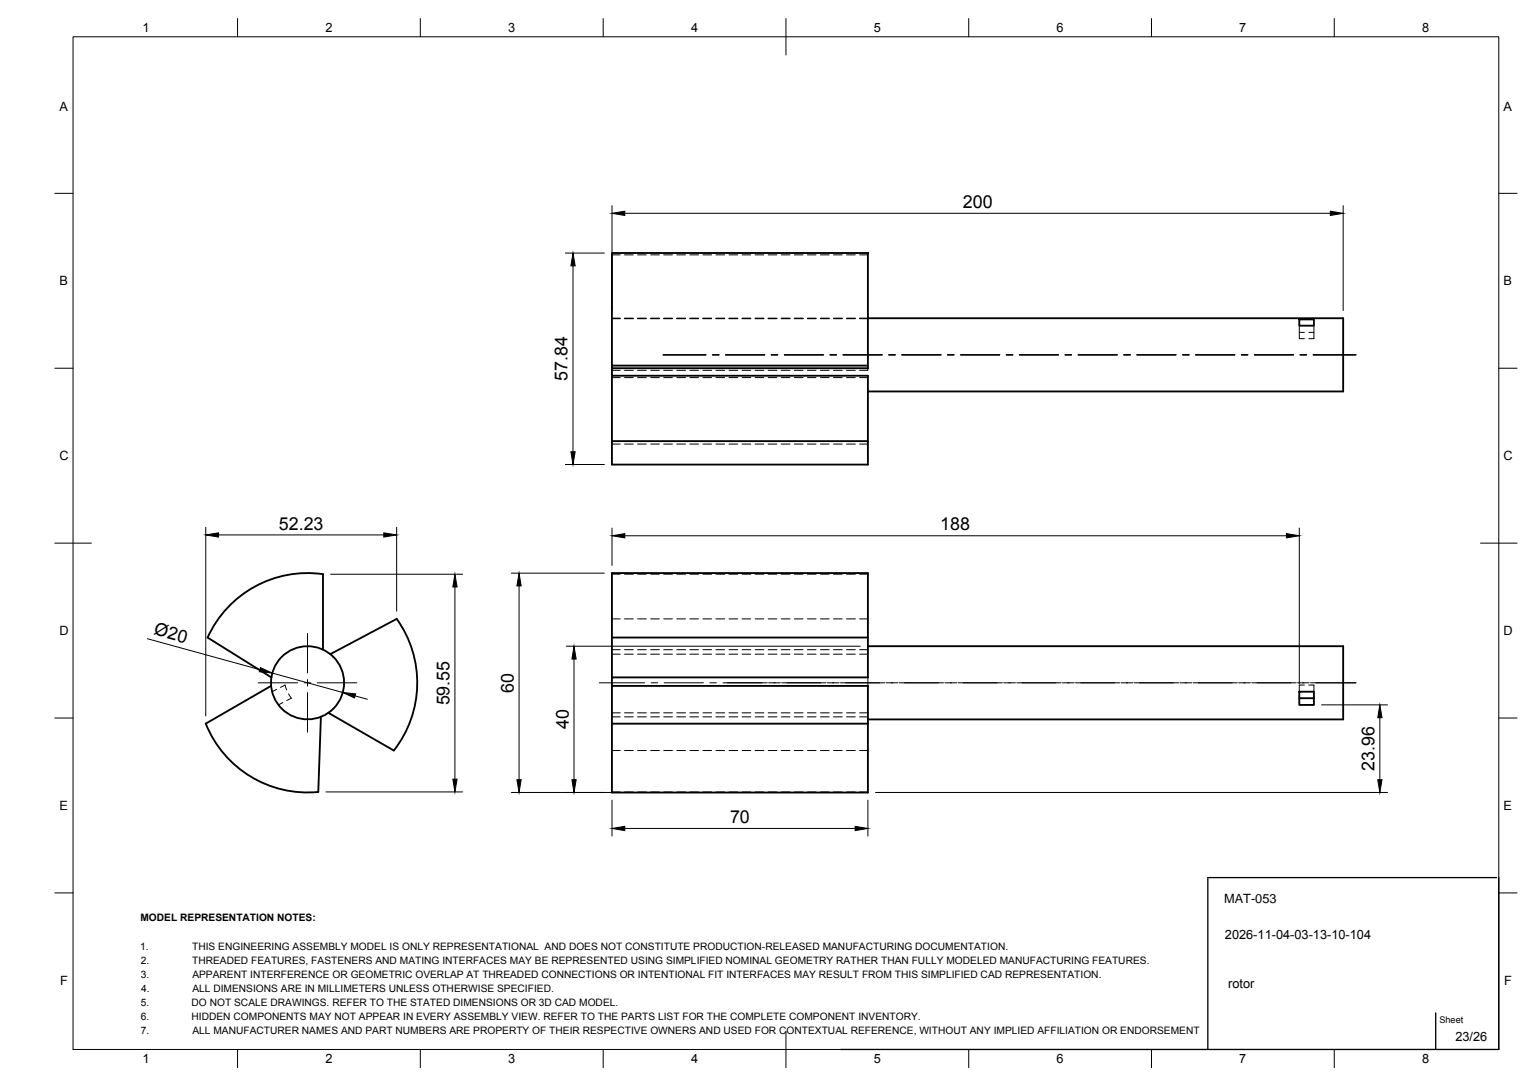
ISO-10303-21;
HEADER;
FILE_DESCRIPTION (('STEP AP214'),
    '1' );
FILE_NAME ('rotor.step',
    '2026-10-10T03:43:58',
    ( '' ),
    ( '' ),
    'SwSTEP 2.0',
    'SolidWorks 2026',
    '' );
FILE_SCHEMA (( 'AUTOMOTIVE_DESIGN' ));
ENDSEC;

DATA;
#17=CARTESIAN_POINT ( 'NONE',  ( 0.000000000000000000, 70.00000000000000000, 0.000000000000000000 ) ) ;
#158=VECTOR ( 'NONE', #16298, 1000.000000000000000 ) ;
#309=LINE ( 'NONE', #37951, #56611 ) ;
#450=VECTOR ( 'NONE', #55912, 1000.000000000000000 ) ;
#456=COLOUR_RGB ( '',0.7921568627450980005, 0.8196078431372548767, 0.9333333333333333481 ) ;
#467=CIRCLE ( 'NONE', #25205, 10.00000000000000000 ) ;
#513=( NAMED_UNIT ( * ) PLANE_ANGLE_UNIT ( ) SI_UNIT ( $, .RADIAN. ) );
#637=ORIENTED_EDGE ( 'NONE', *, *, #53348, .T. ) ;
#947=CARTESIAN_POINT ( 'NONE',  ( 0.000000000000000000, 70.00000000000000000, 0.000000000000000000 ) ) ;
#1209=EDGE_CURVE ( 'NONE', #16807, #23774, #1533, .T. ) ;
#1274=FACE_OUTER_BOUND ( 'NONE', #43238, .T. ) ;
#1425=AXIS2_PLACEMENT_3D ( 'NONE', #25627, #58986, #15401 ) ;
#1533=LINE ( 'NONE', #38469, #44099 ) ;
#1588=CARTESIAN_POINT ( 'NONE',  ( -12.50012419267789454, 70.00000000000000000, -27.27172336262650987 ) ) ;
#1598=FACE_OUTER_BOUND ( 'NONE', #21651, .T. ) ;
#1621=CARTESIAN_POINT ( 'NONE',  ( 0.000000000000000000, 200.0000000000000000, 0.000000000000000000 ) ) ;
#1632=ORIENTED_EDGE ( 'NONE', *, *, #41608, .F. ) ;
#1645=ORIENTED_EDGE ( 'NONE', *, *, #47561, .T. ) ;
#1859=VERTEX_POINT ( 'NONE', #41000 ) ;
#1935=AXIS2_PLACEMENT_3D ( 'NONE', #55616, #50350, #54908 ) ;
#2096=ORIENTED_EDGE ( 'NONE', *, *, #47172, .F. ) ;
#2200=CARTESIAN_POINT ( 'NONE',  ( 0.000000000000000000, 0.000000000000000000, 0.000000000000000000 ) ) ;
#2470=PLANE ( 'NONE',  #7800 ) ;
#2490=PLANE ( 'NONE',  #35776 ) ;
#2533=CIRCLE ( 'NONE', #56453, 30.00000000000000000 ) ;
#2546=ORIENTED_EDGE ( 'NONE', *, *, #59775, .T. ) ;
#2559=EDGE_LOOP ( 'NONE', ( #62181, #13017, #69406, #67367 ) ) ;
#2584=ORIENTED_EDGE ( 'NONE', *, *, #47172, .T. ) ;
#2625=ORIENTED_EDGE ( 'NONE', *, *, #31517, .T. ) ;
#2755=FACE_BOUND ( 'NONE', #28802, .T. ) ;
#2940=CARTESIAN_POINT ( 'NONE',  ( 9.737557066527559257, 192.0000000000000000, 2.275957463600584596 ) ) ;
#3029=EDGE_CURVE ( 'NONE', #41495, #19589, #60995, .T. ) ;
#3127=VECTOR ( 'NONE', #17134, 1000.000000000000000 ) ;
#3205=EDGE_CURVE ( 'NONE', #15244, #53408, #69376, .T. ) ;
#3229=CIRCLE ( 'NONE', #31340, 30.00000000000000000 ) ;
#3559=ADVANCED_FACE ( 'NONE', ( #18572 ), #60439, .F. ) ;
#3584=CYLINDRICAL_SURFACE ( 'NONE', #18065, 30.00000000000000000 ) ;
#3606=DIRECTION ( 'NONE',  ( -0.000000000000000000, 1.000000000000000000, 0.000000000000000000 ) ) ;
#3647=FACE_OUTER_BOUND ( 'NONE', #22136, .T. ) ;
#3725=( GEOMETRIC_REPRESENTATION_CONTEXT ( 3 ) GLOBAL_UNCERTAINTY_ASSIGNED_CONTEXT ( ( #66987 ) ) GLOBAL_UNIT_ASSIGNED_CONTEXT ( ( #56756, #15223, #36690 ) ) REPRESENTATION_CONTEXT ( 'NONE', 'WORKASPACE' ) );
#3943=DIRECTION ( 'NONE',  ( -0.8410447872859948548, 0.000000000000000000, 0.5409654940743040541 ) ) ;
#3944=AXIS2_PLACEMENT_3D ( 'NONE', #67199, #40779, #62236 ) ;
#3990=VECTOR ( 'NONE', #9870, 1000.000000000000000 ) ;
#4513=DIRECTION ( 'NONE',  ( 0.000000000000000000, 0.000000000000000000, -1.000000000000000000 ) ) ;
#4695=CARTESIAN_POINT ( 'NONE',  ( 9.737557066527559257, 188.0000000000000000, 2.275957463600585040 ) ) ;
#4837=CARTESIAN_POINT ( 'NONE',  ( 0.2033771190674383833, 0.000000000000000000, 4.235016458833691821 ) ) ;
#4881=VECTOR ( 'NONE', #9082, 1000.000000000000114 ) ;
#5095=ORIENTED_EDGE ( 'NONE', *, *, #20108, .T. ) ;
#5142=DIRECTION ( 'NONE',  ( 0.000000000000000000, 0.000000000000000000, -1.000000000000000000 ) ) ;
#5186=VECTOR ( 'NONE', #48521, 1000.000000000000000 ) ;
#5268=EDGE_CURVE ( 'NONE', #22494, #32164, #467, .T. ) ;
#5688=AXIS2_PLACEMENT_3D ( 'NONE', #62242, #23924, #39755 ) ;
#5807=PLANE ( 'NONE',  #12101 ) ;
#5820=FACE_OUTER_BOUND ( 'NONE', #11195, .T. ) ;
#5922=CIRCLE ( 'NONE', #32905, 10.00000000000000000 ) ;
#5931=EDGE_CURVE ( 'NONE', #43885, #57004, #38522, .T. ) ;
#5947=FACE_OUTER_BOUND ( 'NONE', #36620, .T. ) ;
#6067=ORIENTED_EDGE ( 'NONE', *, *, #59775, .F. ) ;
#6088=ORIENTED_EDGE ( 'NONE', *, *, #65385, .T. ) ;
#6211=CARTESIAN_POINT ( 'NONE',  ( 9.737557066527559257, 192.0000000000000000, 2.275957463600585040 ) ) ;
#6261=LINE ( 'NONE', #28414, #36185 ) ;
#6269=EDGE_CURVE ( 'NONE', #24463, #24269, #18512, .T. ) ;
#6455=EDGE_CURVE ( 'NONE', #24735, #28455, #61192, .T. ) ;
#6554=DIRECTION ( 'NONE',  ( 0.000000000000000000, -0.000000000000000000, 1.000000000000000000 ) ) ;
#6584=EDGE_CURVE ( 'NONE', #24735, #41495, #13935, .T. ) ;
#6671=CARTESIAN_POINT ( 'NONE',  ( -9.119248870808011276, 0.000000000000000000, 4.103571619000548232 ) ) ;
#6698=CARTESIAN_POINT ( 'NONE',  ( -17.36794314067741496, 70.00000000000000000, 24.46128678263259815 ) ) ;
#6858=ORIENTED_EDGE ( 'NONE', *, *, #8268, .F. ) ;
#7138=VECTOR ( 'NONE', #50452, 1000.000000000000000 ) ;
#7268=VECTOR ( 'NONE', #48702, 1000.000000000000000 ) ;
#7376=EDGE_LOOP ( 'NONE', ( #17858, #25912, #30020, #37099 ) ) ;
#7467=CARTESIAN_POINT ( 'NONE',  ( 18.62350602913453201, 0.000000000000000000, 23.51946052065798298 ) ) ;
#7577=CARTESIAN_POINT ( 'NONE',  ( 0.000000000000000000, 0.000000000000000000, 0.000000000000000000 ) ) ;
#7619=VERTEX_POINT ( 'NONE', #18144 ) ;
#7684=ORIENTED_EDGE ( 'NONE', *, *, #20480, .T. ) ;
#7800=AXIS2_PLACEMENT_3D ( 'NONE', #47017, #41741, #61888 ) ;
#7829=CYLINDRICAL_SURFACE ( 'NONE', #28638, 30.00000000000000000 ) ;
#7957=DIRECTION ( 'NONE',  ( -0.000000000000000000, 1.000000000000000000, -0.000000000000000000 ) ) ;
#8251=ORIENTED_EDGE ( 'NONE', *, *, #19759, .T. ) ;
#8268=EDGE_CURVE ( 'NONE', #8643, #36732, #63662, .T. ) ;
#8319=DIRECTION ( 'NONE',  ( 1.000000000000000000, 0.000000000000000000, 0.000000000000000000 ) ) ;
#8362=MECHANICAL_DESIGN_GEOMETRIC_PRESENTATION_REPRESENTATION('',(#39786),#3725);
#8384=DIRECTION ( 'NONE',  ( -0.000000000000000000, -1.000000000000000000, -0.000000000000000000 ) ) ;
#8517=CARTESIAN_POINT ( 'NONE',  ( 1.224646799147353256E-15, 200.0000000000000000, 10.00000000000000000 ) ) ;
#8543=VERTEX_POINT ( 'NONE', #25611 ) ;
#8643=VERTEX_POINT ( 'NONE', #67319 ) ;
#8758=LINE ( 'NONE', #29499, #68982 ) ;
#8847=PLANE ( 'NONE',  #53612 ) ;
#9082=DIRECTION ( 'NONE',  ( 0.4887922226926450509, 0.000000000000000000, -0.8724002309921654597 ) ) ;
#9354=AXIS2_PLACEMENT_3D ( 'NONE', #45077, #60911, #12734 ) ;
#9450=DIRECTION ( 'NONE',  ( 0.000000000000000000, -1.000000000000000000, 0.000000000000000000 ) ) ;
#9699=LINE ( 'NONE', #15316, #18300 ) ;
#9760=CARTESIAN_POINT ( 'NONE',  ( -9.119248870808011276, 70.00000000000000000, 4.103571619000548232 ) ) ;
#9806=CIRCLE ( 'NONE', #1935, 10.00000000000000000 ) ;
#9808=VERTEX_POINT ( 'NONE', #22364 ) ;
#9870=DIRECTION ( 'NONE',  ( 0.5111246509603011301, 0.000000000000000000, 0.8595065975201763298 ) ) ;
#9984=DIRECTION ( 'NONE',  ( 0.8660254037844433705, 0.000000000000000000, -0.4999999999999918954 ) ) ;
#10072=ORIENTED_EDGE ( 'NONE', *, *, #55049, .T. ) ;
#10118=LINE ( 'NONE', #4837, #34031 ) ;
#10295=AXIS2_PLACEMENT_3D ( 'NONE', #15592, #52853, #58479 ) ;
#10688=ORIENTED_EDGE ( 'NONE', *, *, #6269, .T. ) ;
#10694=AXIS2_PLACEMENT_3D ( 'NONE', #41357, #62809, #14614 ) ;
#10699=ORIENTED_EDGE ( 'NONE', *, *, #32324, .F. ) ;
#10743=FACE_OUTER_BOUND ( 'NONE', #34044, .T. ) ;
#10903=LINE ( 'NONE', #64367, #49186 ) ;
#10960=ADVANCED_FACE ( 'NONE', ( #1274 ), #17086, .T. ) ;
#11102=DIRECTION ( 'NONE',  ( -0.9999168736529502333, 0.000000000000000000, 0.01289363347198224652 ) ) ;
#11175=ORIENTED_EDGE ( 'NONE', *, *, #35410, .T. ) ;
#11187=VECTOR ( 'NONE', #67603, 1000.000000000000000 ) ;
#11195=EDGE_LOOP ( 'NONE', ( #43138, #50240, #35379, #36120, #11963, #1632, #41191, #63277, #68258, #42912 ) ) ;
#11806=( GEOMETRIC_REPRESENTATION_CONTEXT ( 3 ) GLOBAL_UNCERTAINTY_ASSIGNED_CONTEXT ( ( #39538 ) ) GLOBAL_UNIT_ASSIGNED_CONTEXT ( ( #37800, #513, #38141 ) ) REPRESENTATION_CONTEXT ( 'NONE', 'WORKASPACE' ) );
#11963=ORIENTED_EDGE ( 'NONE', *, *, #22370, .T. ) ;
#12101=AXIS2_PLACEMENT_3D ( 'NONE', #31864, #64208, #26585 ) ;
#12156=ORIENTED_EDGE ( 'NONE', *, *, #53282, .F. ) ;
#12160=CARTESIAN_POINT ( 'NONE',  ( -29.68020330876228385, 0.000000000000000000, 4.368699068434031219 ) ) ;
#12734=DIRECTION ( 'NONE',  ( 0.000000000000000000, 0.000000000000000000, -1.000000000000000000 ) ) ;
#12756=CARTESIAN_POINT ( 'NONE',  ( 0.000000000000000000, 70.00000000000000000, 0.000000000000000000 ) ) ;
#12971=DIRECTION ( 'NONE',  ( 0.000000000000000000, 0.000000000000000000, -1.000000000000000000 ) ) ;
#13017=ORIENTED_EDGE ( 'NONE', *, *, #59463, .T. ) ;
#13419=EDGE_CURVE ( 'NONE', #32766, #41495, #62864, .T. ) ;
#13492=DIRECTION ( 'NONE',  ( 0.000000000000000000, -0.000000000000000000, -1.000000000000000000 ) ) ;
#13577=DIRECTION ( 'NONE',  ( -0.000000000000000000, -1.000000000000000000, -0.000000000000000000 ) ) ;
#13604=ORIENTED_EDGE ( 'NONE', *, *, #22162, .F. ) ;
#13935=LINE ( 'NONE', #36782, #34286 ) ;
#13961=EDGE_CURVE ( 'NONE', #18376, #21875, #28435, .T. ) ;
#14150=PLANE ( 'NONE',  #20788 ) ;
#14262=ORIENTED_EDGE ( 'NONE', *, *, #52512, .F. ) ;
#14534=FILL_AREA_STYLE_COLOUR ( '', #456 ) ;
#14614=DIRECTION ( 'NONE',  ( 0.000000000000000000, 0.000000000000000000, -1.000000000000000000 ) ) ;
#14719=FACE_OUTER_BOUND ( 'NONE', #15340, .T. ) ;
#14822=VECTOR ( 'NONE', #60512, 1000.000000000000000 ) ;
#14870=SURFACE_STYLE_FILL_AREA ( #35991 ) ;
#14908=CARTESIAN_POINT ( 'NONE',  ( 9.737557066527559257, 188.0000000000000000, 2.275957463600584596 ) ) ;
#15042=ORIENTED_EDGE ( 'NONE', *, *, #54768, .T. ) ;
#15142=CARTESIAN_POINT ( 'NONE',  ( 18.62350602913453557, 70.00000000000000000, 23.51946052065799364 ) ) ;
#15180=EDGE_CURVE ( 'NONE', #57004, #9808, #53700, .T. ) ;
#15223=( NAMED_UNIT ( * ) PLANE_ANGLE_UNIT ( ) SI_UNIT ( $, .RADIAN. ) );
#15244=VERTEX_POINT ( 'NONE', #32268 ) ;
#15259=DIRECTION ( 'NONE',  ( 0.000000000000000000, -1.000000000000000000, 0.000000000000000000 ) ) ;
#15316=CARTESIAN_POINT ( 'NONE',  ( 0.000000000000000000, 200.0000000000000000, -10.00000000000000000 ) ) ;
#15340=EDGE_LOOP ( 'NONE', ( #65390, #64020, #51418, #38157 ) ) ;
#15401=DIRECTION ( 'NONE',  ( -1.000000000000000000, 0.000000000000000000, -0.000000000000000000 ) ) ;
#15472=CIRCLE ( 'NONE', #33452, 10.00000000000000000 ) ;
#15592=CARTESIAN_POINT ( 'NONE',  ( 9.737557066527559257, 200.0000000000000000, 2.275957463600584596 ) ) ;
#15661=DIRECTION ( 'NONE',  ( -0.000000000000000000, -1.000000000000000000, -0.000000000000000000 ) ) ;
#15663=DIRECTION ( 'NONE',  ( 0.000000000000000000, -1.000000000000000000, 0.000000000000000000 ) ) ;
#15702=VECTOR ( 'NONE', #66791, 1000.000000000000000 ) ;
#15713=ORIENTED_EDGE ( 'NONE', *, *, #6455, .T. ) ;
#16298=DIRECTION ( 'NONE',  ( -1.000000000000000000, 0.000000000000000000, 0.000000000000000000 ) ) ;
#16595=ORIENTED_EDGE ( 'NONE', *, *, #31517, .F. ) ;
#16661=ORIENTED_EDGE ( 'NONE', *, *, #59463, .F. ) ;
#16742=ORIENTED_EDGE ( 'NONE', *, *, #24162, .F. ) ;
#16807=VERTEX_POINT ( 'NONE', #53772 ) ;
#16822=ORIENTED_EDGE ( 'NONE', *, *, #45120, .T. ) ;
#16837=ORIENTED_EDGE ( 'NONE', *, *, #53571, .F. ) ;
#17075=AXIS2_PLACEMENT_3D ( 'NONE', #18933, #8384, #12971 ) ;
#17086=PLANE ( 'NONE',  #52536 ) ;
#17095=EDGE_LOOP ( 'NONE', ( #52386, #18112, #28006, #32395 ) ) ;
#17103=DIRECTION ( 'NONE',  ( -0.8660254037844362651, 0.000000000000000000, -0.5000000000000038858 ) ) ;
#17134=DIRECTION ( 'NONE',  ( -0.000000000000000000, 1.000000000000000000, -0.000000000000000000 ) ) ;
#17242=EDGE_LOOP ( 'NONE', ( #52824, #58022, #67424, #2546 ) ) ;
#17320=ORIENTED_EDGE ( 'NONE', *, *, #13419, .F. ) ;
#17348=DIRECTION ( 'NONE',  ( 0.000000000000000000, -1.000000000000000000, 0.000000000000000000 ) ) ;
#17365=VERTEX_POINT ( 'NONE', #28271 ) ;
#17466=CARTESIAN_POINT ( 'NONE',  ( -29.68020330876228030, 0.000000000000000000, 4.368699068434031219 ) ) ;
#17492=CARTESIAN_POINT ( 'NONE',  ( 1.224646799147353256E-15, 200.0000000000000000, 10.00000000000000000 ) ) ;
#17691=ORIENTED_EDGE ( 'NONE', *, *, #55587, .T. ) ;
#17858=ORIENTED_EDGE ( 'NONE', *, *, #53236, .F. ) ;
#17892=CARTESIAN_POINT ( 'NONE',  ( 0.000000000000000000, 70.00000000000000000, 0.000000000000000000 ) ) ;
#17900=DIRECTION ( 'NONE',  ( -1.000000000000000000, 0.000000000000000000, 0.000000000000000000 ) ) ;
#18009=CARTESIAN_POINT ( 'NONE',  ( 8.113421703707349053, 70.00000000000000000, 5.845715376051984435 ) ) ;
#18065=AXIS2_PLACEMENT_3D ( 'NONE', #46487, #58088, #27100 ) ;
#18112=ORIENTED_EDGE ( 'NONE', *, *, #3029, .F. ) ;
#18144=CARTESIAN_POINT ( 'NONE',  ( 29.86806733335506436, 70.00000000000000000, 2.810436579993893957 ) ) ;
#18265=EDGE_CURVE ( 'NONE', #27416, #21875, #30226, .T. ) ;
#18300=VECTOR ( 'NONE', #15661, 1000.000000000000000 ) ;
#18376=VERTEX_POINT ( 'NONE', #62581 ) ;
#18512=CIRCLE ( 'NONE', #48798, 30.00000000000000000 ) ;
#18572=FACE_OUTER_BOUND ( 'NONE', #17242, .T. ) ;
#18600=AXIS2_PLACEMENT_3D ( 'NONE', #43927, #54482, #27407 ) ;
#18683=FACE_OUTER_BOUND ( 'NONE', #37789, .T. ) ;
#18749=LINE ( 'NONE', #40207, #63574 ) ;
#18826=ORIENTED_EDGE ( 'NONE', *, *, #25756, .T. ) ;
#18933=CARTESIAN_POINT ( 'NONE',  ( 0.000000000000000000, 200.0000000000000000, 0.000000000000000000 ) ) ;
#18937=VERTEX_POINT ( 'NONE', #52862 ) ;
#19410=AXIS2_PLACEMENT_3D ( 'NONE', #49515, #34422, #38995 ) ;
#19489=CARTESIAN_POINT ( 'NONE',  ( 9.737557066527559257, 200.0000000000000000, 2.275957463600584596 ) ) ;
#19589=VERTEX_POINT ( 'NONE', #48358 ) ;
#19639=DIRECTION ( 'NONE',  ( -1.000000000000000000, 0.000000000000000000, 0.000000000000000000 ) ) ;
#19759=EDGE_CURVE ( 'NONE', #32766, #23774, #21564, .T. ) ;
#19928=ORIENTED_EDGE ( 'NONE', *, *, #69410, .T. ) ;
#20108=EDGE_CURVE ( 'NONE', #24269, #27416, #22180, .T. ) ;
#20308=ORIENTED_EDGE ( 'NONE', *, *, #22057, .F. ) ;
#20480=EDGE_CURVE ( 'NONE', #48193, #58381, #6261, .T. ) ;
#20490=PRESENTATION_STYLE_ASSIGNMENT (( #57446 ) ) ;
#20674=CARTESIAN_POINT ( 'NONE',  ( 5.737557066527558369, 188.0000000000000000, 2.275957463600585040 ) ) ;
#20778=LINE ( 'NONE', #31682, #5186 ) ;
#20788=AXIS2_PLACEMENT_3D ( 'NONE', #40529, #3943, #41914 ) ;
#20839=VERTEX_POINT ( 'NONE', #21757 ) ;
#21094=DIRECTION ( 'NONE',  ( -0.000000000000000000, 1.000000000000000000, -0.000000000000000000 ) ) ;
#21275=EDGE_LOOP ( 'NONE', ( #48937, #6067, #1645, #32059, #28609 ) ) ;
#21564=LINE ( 'NONE', #14908, #158 ) ;
#21575=EDGE_LOOP ( 'NONE', ( #62682, #36983, #35955, #40340 ) ) ;
#21651=EDGE_LOOP ( 'NONE', ( #54885, #45467, #21777, #2625 ) ) ;
#21757=CARTESIAN_POINT ( 'NONE',  ( -1.333402737265964699, 0.000000000000000000, -9.910703160737465822 ) ) ;
#21777=ORIENTED_EDGE ( 'NONE', *, *, #41837, .T. ) ;
#21783=PLANE ( 'NONE',  #18600 ) ;
#21875=VERTEX_POINT ( 'NONE', #31314 ) ;
#21940=EDGE_LOOP ( 'NONE', ( #16661, #20308, #15713, #38662 ) ) ;
#22049=AXIS2_PLACEMENT_3D ( 'NONE', #36182, #58313, #47406 ) ;
#22057=EDGE_CURVE ( 'NONE', #24735, #18937, #28447, .T. ) ;
#22098=DIRECTION ( 'NONE',  ( 0.4887922226926451064, 0.000000000000000000, -0.8724002309921654597 ) ) ;
#22136=EDGE_LOOP ( 'NONE', ( #66291, #30867, #17691, #8251 ) ) ;
#22162=EDGE_CURVE ( 'NONE', #24494, #1859, #36156, .T. ) ;
#22180=LINE ( 'NONE', #6698, #14822 ) ;
#22343=DIRECTION ( 'NONE',  ( 0.000000000000000000, -1.000000000000000000, 0.000000000000000000 ) ) ;
#22364=CARTESIAN_POINT ( 'NONE',  ( -1.333402737265964699, 70.00000000000000000, -9.910703160737465822 ) ) ;
#22370=EDGE_CURVE ( 'NONE', #20839, #9808, #56140, .T. ) ;
#22404=CARTESIAN_POINT ( 'NONE',  ( 0.000000000000000000, 0.000000000000000000, -10.00000000000000000 ) ) ;
#22494=VERTEX_POINT ( 'NONE', #32515 ) ;
#22749=DIRECTION ( 'NONE',  ( 0.000000000000000000, 0.000000000000000000, -1.000000000000000000 ) ) ;
#22869=VECTOR ( 'NONE', #41629, 999.9999999999998863 ) ;
#23387=SHAPE_REPRESENTATION_RELATIONSHIP ( 'NONE' , 'NONE' ,  #36174, #54154 ) ;
#23522=FACE_OUTER_BOUND ( 'NONE', #51607, .T. ) ;
#23700=PLANE ( 'NONE',  #27020 ) ;
#23774=VERTEX_POINT ( 'NONE', #20674 ) ;
#23924=DIRECTION ( 'NONE',  ( -0.000000000000000000, -1.000000000000000000, -0.000000000000000000 ) ) ;
#24027=VECTOR ( 'NONE', #7957, 1000.000000000000000 ) ;
#24094=DIRECTION ( 'NONE',  ( -0.000000000000000000, -1.000000000000000000, -0.000000000000000000 ) ) ;
#24162=EDGE_CURVE ( 'NONE', #48193, #8543, #33104, .T. ) ;
#24269=VERTEX_POINT ( 'NONE', #51147 ) ;
#24436=DIRECTION ( 'NONE',  ( 0.000000000000000000, -0.000000000000000000, 1.000000000000000000 ) ) ;
#24463=VERTEX_POINT ( 'NONE', #7467 ) ;
#24494=VERTEX_POINT ( 'NONE', #27859 ) ;
#24629=FACE_OUTER_BOUND ( 'NONE', #2559, .T. ) ;
#24659=CARTESIAN_POINT ( 'NONE',  ( -21.78980970457817179, 0.000000000000000000, 33.04664611826583354 ) ) ;
#24697=DIRECTION ( 'NONE',  ( 0.000000000000000000, -1.000000000000000000, 0.000000000000000000 ) ) ;
#24716=FACE_OUTER_BOUND ( 'NONE', #59779, .T. ) ;
#24735=VERTEX_POINT ( 'NONE', #52941 ) ;
#24816=ORIENTED_EDGE ( 'NONE', *, *, #24162, .T. ) ;
#25205=AXIS2_PLACEMENT_3D ( 'NONE', #34821, #52026, #41127 ) ;
#25405=ORIENTED_EDGE ( 'NONE', *, *, #53348, .F. ) ;
#25422=DIRECTION ( 'NONE',  ( 0.000000000000000000, -0.000000000000000000, -1.000000000000000000 ) ) ;
#25447=PRODUCT_DEFINITION_FORMATION_WITH_SPECIFIED_SOURCE ( 'ANY', '', #65900, .NOT_KNOWN. ) ;
#25470=LINE ( 'NONE', #46907, #22869 ) ;
#25576=ORIENTED_EDGE ( 'NONE', *, *, #60819, .T. ) ;
#25611=CARTESIAN_POINT ( 'NONE',  ( 9.249622075198342230, 70.00000000000000000, 3.800590936420744193 ) ) ;
#25627=CARTESIAN_POINT ( 'NONE',  ( 9.850262805259839993, 200.0000000000000000, -1.724042536399416070 ) ) ;
#25756=EDGE_CURVE ( 'NONE', #43631, #8543, #20778, .T. ) ;
#25829=DIRECTION ( 'NONE',  ( 0.000000000000000000, -1.000000000000000000, 0.000000000000000000 ) ) ;
#25843=ORIENTED_EDGE ( 'NONE', *, *, #5931, .F. ) ;
#25912=ORIENTED_EDGE ( 'NONE', *, *, #19759, .F. ) ;
#26222=CIRCLE ( 'NONE', #9354, 10.00000000000000000 ) ;
#26428=CIRCLE ( 'NONE', #10694, 10.00000000000000000 ) ;
#26442=ADVANCED_FACE ( 'NONE', ( #33863 ), #7829, .T. ) ;
#26585=DIRECTION ( 'NONE',  ( 0.000000000000000000, -0.000000000000000000, -1.000000000000000000 ) ) ;
#26601=CARTESIAN_POINT ( 'NONE',  ( 0.000000000000000000, 200.0000000000000000, 0.000000000000000000 ) ) ;
#26749=ORIENTED_EDGE ( 'NONE', *, *, #22162, .T. ) ;
#27020=AXIS2_PLACEMENT_3D ( 'NONE', #2940, #61673, #13492 ) ;
#27100=DIRECTION ( 'NONE',  ( 0.000000000000000000, 0.000000000000000000, -1.000000000000000000 ) ) ;
#27407=DIRECTION ( 'NONE',  ( 0.000000000000000000, -0.000000000000000000, -1.000000000000000000 ) ) ;
#27416=VERTEX_POINT ( 'NONE', #55697 ) ;
#27575=AXIS2_PLACEMENT_3D ( 'NONE', #26601, #37844, #5142 ) ;
#27668=AXIS2_PLACEMENT_3D ( 'NONE', #41804, #9450, #4513 ) ;
#27709=ADVANCED_FACE ( 'NONE', ( #18683 ), #61918, .F. ) ;
#27859=CARTESIAN_POINT ( 'NONE',  ( 1.005827167100601827, 0.000000000000000000, -9.949286995052577964 ) ) ;
#27967=AXIS2_PLACEMENT_3D ( 'NONE', #7577, #15259, #9984 ) ;
#28006=ORIENTED_EDGE ( 'NONE', *, *, #6584, .F. ) ;
#28271=CARTESIAN_POINT ( 'NONE',  ( 29.86806733335506436, 0.000000000000000000, 2.810436579993893957 ) ) ;
#28414=CARTESIAN_POINT ( 'NONE',  ( 11.05669727962760085, 70.00000000000000000, -27.88815958909220782 ) ) ;
#28435=LINE ( 'NONE', #34073, #15702 ) ;
#28447=LINE ( 'NONE', #49895, #37461 ) ;
#28455=VERTEX_POINT ( 'NONE', #6211 ) ;
#28609=ORIENTED_EDGE ( 'NONE', *, *, #18265, .F. ) ;
#28638=AXIS2_PLACEMENT_3D ( 'NONE', #12756, #44766, #66932 ) ;
#28651=VECTOR ( 'NONE', #58634, 1000.000000000000114 ) ;
#28802=EDGE_LOOP ( 'NONE', ( #60168, #31437, #17320, #48393 ) ) ;
#29313=EDGE_LOOP ( 'NONE', ( #16822, #13604, #10072, #7684 ) ) ;
#29441=CARTESIAN_POINT ( 'NONE',  ( 29.86806733335506792, 70.00000000000000000, 2.810436579993894401 ) ) ;
#29499=CARTESIAN_POINT ( 'NONE',  ( 9.737557066527559257, 192.0000000000000000, 2.275957463600584596 ) ) ;
#29992=ORIENTED_EDGE ( 'NONE', *, *, #31278, .T. ) ;
#30020=ORIENTED_EDGE ( 'NONE', *, *, #13419, .T. ) ;
#30226=LINE ( 'NONE', #35847, #41813 ) ;
#30328=ADVANCED_FACE ( 'NONE', ( #66907 ), #8847, .F. ) ;
#30338=CIRCLE ( 'NONE', #59490, 30.00000000000000000 ) ;
#30522=DIRECTION ( 'NONE',  ( -0.000000000000000000, -1.000000000000000000, -0.000000000000000000 ) ) ;
#30687=FACE_OUTER_BOUND ( 'NONE', #21275, .T. ) ;
#30867=ORIENTED_EDGE ( 'NONE', *, *, #40848, .F. ) ;
#31038=PLANE ( 'NONE',  #40023 ) ;
#31202=VECTOR ( 'NONE', #44836, 1000.000000000000000 ) ;
#31245=DIRECTION ( 'NONE',  ( -0.000000000000000000, 1.000000000000000000, 0.000000000000000000 ) ) ;
#31278=EDGE_CURVE ( 'NONE', #24269, #18376, #46209, .T. ) ;
#31314=CARTESIAN_POINT ( 'NONE',  ( -7.916219337932451694, 70.00000000000000000, 6.110112224316693208 ) ) ;
#31330=DIRECTION ( 'NONE',  ( 0.000000000000000000, -1.000000000000000000, 0.000000000000000000 ) ) ;
#31340=AXIS2_PLACEMENT_3D ( 'NONE', #32894, #22343, #43437 ) ;
#31437=ORIENTED_EDGE ( 'NONE', *, *, #6584, .T. ) ;
#31517=EDGE_CURVE ( 'NONE', #46033, #37671, #10903, .T. ) ;
#31682=CARTESIAN_POINT ( 'NONE',  ( 9.249622075198342230, 0.000000000000000000, 3.800590936420744193 ) ) ;
#31864=CARTESIAN_POINT ( 'NONE',  ( 0.000000000000000000, 70.00000000000000000, 0.000000000000000000 ) ) ;
#31925=LINE ( 'NONE', #48078, #28651 ) ;
#31926=VERTEX_POINT ( 'NONE', #48103 ) ;
#31965=CARTESIAN_POINT ( 'NONE',  ( 8.113421703707349053, 0.000000000000000000, 5.845715376051984435 ) ) ;
#32059=ORIENTED_EDGE ( 'NONE', *, *, #46537, .T. ) ;
#32164=VERTEX_POINT ( 'NONE', #17492 ) ;
#32268=CARTESIAN_POINT ( 'NONE',  ( -9.119248870808011276, 0.000000000000000000, 4.103571619000548232 ) ) ;
#32324=EDGE_CURVE ( 'NONE', #37671, #57004, #3229, .T. ) ;
#32395=ORIENTED_EDGE ( 'NONE', *, *, #22057, .T. ) ;
#32442=PRODUCT_DEFINITION_CONTEXT ( 'detailed design', #51204, 'design' ) ;
#32515=CARTESIAN_POINT ( 'NONE',  ( 0.000000000000000000, 200.0000000000000000, -10.00000000000000000 ) ) ;
#32607=CARTESIAN_POINT ( 'NONE',  ( -17.72433019600386217, 70.00000000000000000, -35.39385180692614341 ) ) ;
#32653=EDGE_CURVE ( 'NONE', #18376, #15244, #45950, .T. ) ;
#32766=VERTEX_POINT ( 'NONE', #4695 ) ;
#32894=CARTESIAN_POINT ( 'NONE',  ( 0.000000000000000000, 70.00000000000000000, 0.000000000000000000 ) ) ;
#32905=AXIS2_PLACEMENT_3D ( 'NONE', #38947, #39289, #39629 ) ;
#33030=ADVANCED_FACE ( 'NONE', ( #50647 ), #2470, .F. ) ;
#33104=CIRCLE ( 'NONE', #55598, 10.00000000000000000 ) ;
#33209=AXIS2_PLACEMENT_3D ( 'NONE', #24659, #57009, #46437 ) ;
#33367=AXIS2_PLACEMENT_3D ( 'NONE', #52188, #56783, #24436 ) ;
#33428=ORIENTED_EDGE ( 'NONE', *, *, #5268, .T. ) ;
#33452=AXIS2_PLACEMENT_3D ( 'NONE', #947, #31330, #22749 ) ;
#33659=CARTESIAN_POINT ( 'NONE',  ( -1.333402737265964699, 0.000000000000000000, -9.910703160737465822 ) ) ;
#33863=FACE_OUTER_BOUND ( 'NONE', #21575, .T. ) ;
#34031=VECTOR ( 'NONE', #52675, 1000.000000000000114 ) ;
#34044=EDGE_LOOP ( 'NONE', ( #10699, #16595, #61976, #38311 ) ) ;
#34073=CARTESIAN_POINT ( 'NONE',  ( -7.916219337932451694, 0.000000000000000000, 6.110112224316693208 ) ) ;
#34250=ORIENTED_EDGE ( 'NONE', *, *, #13961, .F. ) ;
#34286=VECTOR ( 'NONE', #58225, 1000.000000000000000 ) ;
#34422=DIRECTION ( 'NONE',  ( -0.8595065975201763298, 0.000000000000000000, 0.5111246509603011301 ) ) ;
#34515=FACE_OUTER_BOUND ( 'NONE', #7376, .T. ) ;
#34540=ORIENTED_EDGE ( 'NONE', *, *, #5931, .T. ) ;
#34572=CIRCLE ( 'NONE', #43519, 30.00000000000000000 ) ;
#34637=LINE ( 'NONE', #62033, #7138 ) ;
#34773=DIRECTION ( 'NONE',  ( 0.000000000000000000, 0.000000000000000000, -1.000000000000000000 ) ) ;
#34821=CARTESIAN_POINT ( 'NONE',  ( 0.000000000000000000, 200.0000000000000000, 0.000000000000000000 ) ) ;
#35234=LINE ( 'NONE', #46127, #63345 ) ;
#35379=ORIENTED_EDGE ( 'NONE', *, *, #53571, .T. ) ;
#35410=EDGE_CURVE ( 'NONE', #20839, #53439, #57318, .T. ) ;
#35491=CYLINDRICAL_SURFACE ( 'NONE', #27668, 30.00000000000000000 ) ;
#35776=AXIS2_PLACEMENT_3D ( 'NONE', #40123, #61580, #55959 ) ;
#35847=CARTESIAN_POINT ( 'NONE',  ( -21.78980970457817179, 70.00000000000000000, 33.04664611826583354 ) ) ;
#35902=AXIS2_PLACEMENT_3D ( 'NONE', #40543, #3606, #49436 ) ;
#35955=ORIENTED_EDGE ( 'NONE', *, *, #45120, .F. ) ;
#35991=FILL_AREA_STYLE ('',( #14534 ) ) ;
#36004=CARTESIAN_POINT ( 'NONE',  ( 9.850262805259839993, 188.0000000000000000, -1.724042536399416070 ) ) ;
#36053=ADVANCED_FACE ( 'NONE', ( #40224 ), #23700, .T. ) ;
#36120=ORIENTED_EDGE ( 'NONE', *, *, #35410, .F. ) ;
#36156=LINE ( 'NONE', #62550, #4881 ) ;
#36174=SHAPE_REPRESENTATION ( 'rotor', ( #66832 ), #11806 ) ;
#36182=CARTESIAN_POINT ( 'NONE',  ( 0.000000000000000000, 0.000000000000000000, 0.000000000000000000 ) ) ;
#36185=VECTOR ( 'NONE', #22098, 1000.000000000000000 ) ;
#36620=EDGE_LOOP ( 'NONE', ( #24816, #41353, #14262, #59290 ) ) ;
#36690=( NAMED_UNIT ( * ) SI_UNIT ( $, .STERADIAN. ) SOLID_ANGLE_UNIT ( ) );
#36732=VERTEX_POINT ( 'NONE', #18009 ) ;
#36782=CARTESIAN_POINT ( 'NONE',  ( 9.850262805259839993, 200.0000000000000000, -1.724042536399416070 ) ) ;
#36983=ORIENTED_EDGE ( 'NONE', *, *, #65385, .F. ) ;
#37021=LINE ( 'NONE', #53523, #63344 ) ;
#37099=ORIENTED_EDGE ( 'NONE', *, *, #3029, .T. ) ;
#37111=DIRECTION ( 'NONE',  ( 0.000000000000000000, 0.000000000000000000, -1.000000000000000000 ) ) ;
#37129=ORIENTED_EDGE ( 'NONE', *, *, #41385, .F. ) ;
#37191=DIRECTION ( 'NONE',  ( 0.000000000000000000, 0.000000000000000000, 1.000000000000000000 ) ) ;
#37408=ADVANCED_FACE ( 'NONE', ( #3647 ), #46552, .T. ) ;
#37461=VECTOR ( 'NONE', #17900, 1000.000000000000000 ) ;
#37659=ORIENTED_EDGE ( 'NONE', *, *, #25756, .F. ) ;
#37671=VERTEX_POINT ( 'NONE', #55289 ) ;
#37708=DIRECTION ( 'NONE',  ( -0.9999168736529502333, 0.000000000000000000, 0.01289363347198229856 ) ) ;
#37789=EDGE_LOOP ( 'NONE', ( #5095, #58886, #34250, #60792 ) ) ;
#37800=( LENGTH_UNIT ( ) NAMED_UNIT ( * ) SI_UNIT ( .MILLI., .METRE. ) );
#37844=DIRECTION ( 'NONE',  ( -0.000000000000000000, -1.000000000000000000, -0.000000000000000000 ) ) ;
#37925=LINE ( 'NONE', #31965, #41003 ) ;
#37951=CARTESIAN_POINT ( 'NONE',  ( 18.62350602913453201, 70.00000000000000000, 23.51946052065798298 ) ) ;
#38141=( NAMED_UNIT ( * ) SI_UNIT ( $, .STERADIAN. ) SOLID_ANGLE_UNIT ( ) );
#38157=ORIENTED_EDGE ( 'NONE', *, *, #6269, .F. ) ;
#38311=ORIENTED_EDGE ( 'NONE', *, *, #15180, .F. ) ;
#38469=CARTESIAN_POINT ( 'NONE',  ( 5.737557066527558369, 200.0000000000000000, 2.275957463600584596 ) ) ;
#38522=LINE ( 'NONE', #1588, #7268 ) ;
#38574=DIRECTION ( 'NONE',  ( 0.5409654940743039431, 0.000000000000000000, 0.8410447872859947438 ) ) ;
#38662=ORIENTED_EDGE ( 'NONE', *, *, #40848, .T. ) ;
#38939=CARTESIAN_POINT ( 'NONE',  ( 0.000000000000000000, 0.000000000000000000, 0.000000000000000000 ) ) ;
#38947=CARTESIAN_POINT ( 'NONE',  ( 0.000000000000000000, 200.0000000000000000, 0.000000000000000000 ) ) ;
#38995=DIRECTION ( 'NONE',  ( 0.5111246509603011301, 0.000000000000000000, 0.8595065975201763298 ) ) ;
#39021=EDGE_CURVE ( 'NONE', #54785, #27416, #2533, .T. ) ;
#39289=DIRECTION ( 'NONE',  ( 0.000000000000000000, 1.000000000000000000, 0.000000000000000000 ) ) ;
#39318=ORIENTED_EDGE ( 'NONE', *, *, #55049, .F. ) ;
#39538=UNCERTAINTY_MEASURE_WITH_UNIT (LENGTH_MEASURE( 1.000000000000000082E-05 ), #37800, 'distance_accuracy_value', 'NONE');
#39629=DIRECTION ( 'NONE',  ( 0.000000000000000000, 0.000000000000000000, 1.000000000000000000 ) ) ;
#39663=ORIENTED_EDGE ( 'NONE', *, *, #47650, .T. ) ;
#39755=DIRECTION ( 'NONE',  ( 0.000000000000000000, 0.000000000000000000, -1.000000000000000000 ) ) ;
#39786=STYLED_ITEM ( 'NONE', ( #20490 ), #40699 ) ;
#39906=CARTESIAN_POINT ( 'NONE',  ( -3.769320398328897870, 0.000000000000000000, -1.941378477755967502 ) ) ;
#39999=LINE ( 'NONE', #29441, #3127 ) ;
#40023=AXIS2_PLACEMENT_3D ( 'NONE', #52137, #41581, #25422 ) ;
#40105=CYLINDRICAL_SURFACE ( 'NONE', #5688, 10.00000000000000000 ) ;
#40123=CARTESIAN_POINT ( 'NONE',  ( 9.850262805259839993, 188.0000000000000000, -1.724042536399416070 ) ) ;
#40207=CARTESIAN_POINT ( 'NONE',  ( 11.05669727962759907, 70.00000000000000000, -27.88815958909220782 ) ) ;
#40224=FACE_OUTER_BOUND ( 'NONE', #21940, .T. ) ;
#40340=ORIENTED_EDGE ( 'NONE', *, *, #52512, .T. ) ;
#40529=CARTESIAN_POINT ( 'NONE',  ( -17.72433019600386217, 0.000000000000000000, -35.39385180692614341 ) ) ;
#40543=CARTESIAN_POINT ( 'NONE',  ( 0.000000000000000000, 188.0000000000000000, 0.000000000000000000 ) ) ;
#40699=MANIFOLD_SOLID_BREP ( 'Cut-Extrude2', #57536 ) ;
#40779=DIRECTION ( 'NONE',  ( 0.000000000000000000, -1.000000000000000000, 0.000000000000000000 ) ) ;
#40818=ORIENTED_EDGE ( 'NONE', *, *, #32653, .T. ) ;
#40848=EDGE_CURVE ( 'NONE', #28455, #16807, #8758, .T. ) ;
#40862=LINE ( 'NONE', #8517, #11187 ) ;
#41000=CARTESIAN_POINT ( 'NONE',  ( 11.05669727962759907, 0.000000000000000000, -27.88815958909220782 ) ) ;
#41003=VECTOR ( 'NONE', #49153, 1000.000000000000114 ) ;
#41127=DIRECTION ( 'NONE',  ( 0.000000000000000000, 0.000000000000000000, 1.000000000000000000 ) ) ;
#41191=ORIENTED_EDGE ( 'NONE', *, *, #41837, .F. ) ;
#41353=ORIENTED_EDGE ( 'NONE', *, *, #69410, .F. ) ;
#41357=CARTESIAN_POINT ( 'NONE',  ( -4.000000000000000000, 192.0000000000000000, 0.000000000000000000 ) ) ;
#41385=EDGE_CURVE ( 'NONE', #37671, #53408, #34637, .T. ) ;
#41495=VERTEX_POINT ( 'NONE', #36004 ) ;
#41581=DIRECTION ( 'NONE',  ( 0.000000000000000000, -1.000000000000000000, 0.000000000000000000 ) ) ;
#41608=EDGE_CURVE ( 'NONE', #46033, #9808, #26222, .T. ) ;
#41629=DIRECTION ( 'NONE',  ( 0.5409654940743039431, -0.000000000000000000, 0.8410447872859948548 ) ) ;
#41741=DIRECTION ( 'NONE',  ( -0.04796746679614544845, 0.000000000000000000, -0.9988488985473031878 ) ) ;
#41804=CARTESIAN_POINT ( 'NONE',  ( 0.000000000000000000, 70.00000000000000000, 0.000000000000000000 ) ) ;
#41813=VECTOR ( 'NONE', #52017, 1000.000000000000000 ) ;
#41837=EDGE_CURVE ( 'NONE', #15244, #46033, #60484, .T. ) ;
#41914=DIRECTION ( 'NONE',  ( 0.5409654940743039431, 0.000000000000000000, 0.8410447872859947438 ) ) ;
#42912=ORIENTED_EDGE ( 'NONE', *, *, #46537, .F. ) ;
#43138=ORIENTED_EDGE ( 'NONE', *, *, #65358, .F. ) ;
#43238=EDGE_LOOP ( 'NONE', ( #33428, #637 ) ) ;
#43437=DIRECTION ( 'NONE',  ( 0.000000000000000000, 0.000000000000000000, -1.000000000000000000 ) ) ;
#43519=AXIS2_PLACEMENT_3D ( 'NONE', #38939, #49106, #60385 ) ;
#43631=VERTEX_POINT ( 'NONE', #56043 ) ;
#43754=ORIENTED_EDGE ( 'NONE', *, *, #49949, .T. ) ;
#43885=VERTEX_POINT ( 'NONE', #69176 ) ;
#43927=CARTESIAN_POINT ( 'NONE',  ( 0.000000000000000000, 70.00000000000000000, 0.000000000000000000 ) ) ;
#44099=VECTOR ( 'NONE', #54280, 1000.000000000000000 ) ;
#44133=ADVANCED_FACE ( 'NONE', ( #24716 ), #14150, .F. ) ;
#44208=ORIENTED_EDGE ( 'NONE', *, *, #57109, .T. ) ;
#44323=EDGE_LOOP ( 'NONE', ( #43754, #19928, #37659, #12156 ) ) ;
#44558=DIRECTION ( 'NONE',  ( 0.000000000000000000, 0.000000000000000000, 1.000000000000000000 ) ) ;
#44766=DIRECTION ( 'NONE',  ( 0.000000000000000000, -1.000000000000000000, 0.000000000000000000 ) ) ;
#44836=DIRECTION ( 'NONE',  ( 0.4578834044730072383, 0.000000000000000000, -0.8890122540821405739 ) ) ;
#44957=AXIS2_PLACEMENT_3D ( 'NONE', #67814, #30522, #46003 ) ;
#45077=CARTESIAN_POINT ( 'NONE',  ( 0.000000000000000000, 70.00000000000000000, 0.000000000000000000 ) ) ;
#45120=EDGE_CURVE ( 'NONE', #58381, #1859, #18749, .T. ) ;
#45154=DIRECTION ( 'NONE',  ( -1.000000000000000000, 0.000000000000000000, 0.000000000000000000 ) ) ;
#45273=ADVANCED_FACE ( 'NONE', ( #30687 ), #31038, .F. ) ;
#45416=VECTOR ( 'NONE', #24094, 1000.000000000000000 ) ;
#45467=ORIENTED_EDGE ( 'NONE', *, *, #3205, .F. ) ;
#45950=CIRCLE ( 'NONE', #27967, 10.00000000000000000 ) ;
#46003=DIRECTION ( 'NONE',  ( 0.000000000000000000, 0.000000000000000000, 1.000000000000000000 ) ) ;
#46033=VERTEX_POINT ( 'NONE', #9760 ) ;
#46104=ORIENTED_EDGE ( 'NONE', *, *, #60819, .F. ) ;
#46127=CARTESIAN_POINT ( 'NONE',  ( 1.005827167100601827, 0.000000000000000000, -9.949286995052577964 ) ) ;
#46209=LINE ( 'NONE', #39906, #31202 ) ;
#46210=PLANE ( 'NONE',  #33367 ) ;
#46367=AXIS2_PLACEMENT_3D ( 'NONE', #53705, #31245, #37191 ) ;
#46437=DIRECTION ( 'NONE',  ( 0.4578834044730072383, 0.000000000000000000, -0.8890122540821405739 ) ) ;
#46487=CARTESIAN_POINT ( 'NONE',  ( 0.000000000000000000, 70.00000000000000000, 0.000000000000000000 ) ) ;
#46537=EDGE_CURVE ( 'NONE', #31926, #21875, #9806, .T. ) ;
#46552=PLANE ( 'NONE',  #10295 ) ;
#46557=FACE_OUTER_BOUND ( 'NONE', #66264, .T. ) ;
#46820=ORIENTED_EDGE ( 'NONE', *, *, #54768, .F. ) ;
#46907=CARTESIAN_POINT ( 'NONE',  ( 3.565943279261457821, 0.000000000000000000, -2.293637981077754073 ) ) ;
#46977=ORIENTED_EDGE ( 'NONE', *, *, #32324, .T. ) ;
#47017=CARTESIAN_POINT ( 'NONE',  ( 39.51413990058172487, 0.000000000000000000, 2.347205688660291667 ) ) ;
#47172=EDGE_CURVE ( 'NONE', #53408, #43885, #34572, .T. ) ;
#47255=DIRECTION ( 'NONE',  ( 0.000000000000000000, 0.000000000000000000, -1.000000000000000000 ) ) ;
#47406=DIRECTION ( 'NONE',  ( 0.000000000000000000, 0.000000000000000000, 1.000000000000000000 ) ) ;
#47561=EDGE_CURVE ( 'NONE', #36732, #31926, #15472, .T. ) ;
#47650=EDGE_CURVE ( 'NONE', #43631, #8643, #54770, .T. ) ;
#47737=PLANE ( 'NONE',  #1425 ) ;
#47851=CIRCLE ( 'NONE', #22049, 10.00000000000000000 ) ;
#48078=CARTESIAN_POINT ( 'NONE',  ( 39.51413990058172487, 70.00000000000000000, 2.347205688660291667 ) ) ;
#48103=CARTESIAN_POINT ( 'NONE',  ( 1.224646799147353256E-15, 70.00000000000000000, 10.00000000000000000 ) ) ;
#48193=VERTEX_POINT ( 'NONE', #59767 ) ;
#48358=CARTESIAN_POINT ( 'NONE',  ( 5.850262805259840881, 188.0000000000000000, -1.724042536399415404 ) ) ;
#48393=ORIENTED_EDGE ( 'NONE', *, *, #55587, .F. ) ;
#48471=CARTESIAN_POINT ( 'NONE',  ( 8.113421703707349053, 0.000000000000000000, 5.845715376051984435 ) ) ;
#48521=DIRECTION ( 'NONE',  ( -0.000000000000000000, 1.000000000000000000, -0.000000000000000000 ) ) ;
#48702=DIRECTION ( 'NONE',  ( -0.000000000000000000, 1.000000000000000000, -0.000000000000000000 ) ) ;
#48798=AXIS2_PLACEMENT_3D ( 'NONE', #52543, #25829, #47255 ) ;
#48937=ORIENTED_EDGE ( 'NONE', *, *, #39021, .F. ) ;
#49106=DIRECTION ( 'NONE',  ( 0.000000000000000000, -1.000000000000000000, 0.000000000000000000 ) ) ;
#49153=DIRECTION ( 'NONE',  ( 0.5111246509603012411, 0.000000000000000000, 0.8595065975201762187 ) ) ;
#49186=VECTOR ( 'NONE', #64726, 1000.000000000000227 ) ;
#49436=DIRECTION ( 'NONE',  ( 0.000000000000000000, 0.000000000000000000, 1.000000000000000000 ) ) ;
#49515=CARTESIAN_POINT ( 'NONE',  ( 18.62350602913453557, 0.000000000000000000, 23.51946052065799364 ) ) ;
#49895=CARTESIAN_POINT ( 'NONE',  ( 9.850262805259839993, 192.0000000000000000, -1.724042536399416070 ) ) ;
#49949=EDGE_CURVE ( 'NONE', #17365, #7619, #39999, .T. ) ;
#50205=ADVANCED_FACE ( 'NONE', ( #10743 ), #5807, .F. ) ;
#50240=ORIENTED_EDGE ( 'NONE', *, *, #5268, .F. ) ;
#50328=ORIENTED_EDGE ( 'NONE', *, *, #53282, .T. ) ;
#50350=DIRECTION ( 'NONE',  ( 0.000000000000000000, -1.000000000000000000, 0.000000000000000000 ) ) ;
#50452=DIRECTION ( 'NONE',  ( 0.000000000000000000, -1.000000000000000000, 0.000000000000000000 ) ) ;
#50530=CARTESIAN_POINT ( 'NONE',  ( 0.000000000000000000, 0.000000000000000000, 0.000000000000000000 ) ) ;
#50639=AXIS2_PLACEMENT_3D ( 'NONE', #12160, #55404, #11102 ) ;
#50647=FACE_OUTER_BOUND ( 'NONE', #44323, .T. ) ;
#50825=ADVANCED_FACE ( 'NONE', ( #1598 ), #65988, .F. ) ;
#51069=DIRECTION ( 'NONE',  ( -0.000000000000000000, 1.000000000000000000, -0.000000000000000000 ) ) ;
#51147=CARTESIAN_POINT ( 'NONE',  ( -17.36794314067741496, 0.000000000000000000, 24.46128678263259815 ) ) ;
#51204=APPLICATION_CONTEXT ( 'automotive_design' ) ;
#51418=ORIENTED_EDGE ( 'NONE', *, *, #20108, .F. ) ;
#51485=SURFACE_SIDE_STYLE ('',( #14870 ) ) ;
#51607=EDGE_LOOP ( 'NONE', ( #25405, #69537, #54241, #6858, #65605, #18826, #16742, #39318, #46104, #16837 ) ) ;
#51611=APPLICATION_CONTEXT ( 'automotive_design' ) ;
#51778=FACE_OUTER_BOUND ( 'NONE', #61527, .T. ) ;
#52003=VECTOR ( 'NONE', #45154, 1000.000000000000000 ) ;
#52017=DIRECTION ( 'NONE',  ( 0.4578834044730071828, 0.000000000000000000, -0.8890122540821405739 ) ) ;
#52026=DIRECTION ( 'NONE',  ( 0.000000000000000000, 1.000000000000000000, 0.000000000000000000 ) ) ;
#52087=DIRECTION ( 'NONE',  ( 0.8724002309921654597, 0.000000000000000000, 0.4887922226926451619 ) ) ;
#52137=CARTESIAN_POINT ( 'NONE',  ( 0.000000000000000000, 70.00000000000000000, 0.000000000000000000 ) ) ;
#52188=CARTESIAN_POINT ( 'NONE',  ( 0.000000000000000000, 0.000000000000000000, 0.000000000000000000 ) ) ;
#52386=ORIENTED_EDGE ( 'NONE', *, *, #68391, .T. ) ;
#52512=EDGE_CURVE ( 'NONE', #58381, #7619, #58659, .T. ) ;
#52521=ADVANCED_FACE ( 'NONE', ( #2755, #23522 ), #60790, .T. ) ;
#52536=AXIS2_PLACEMENT_3D ( 'NONE', #1621, #54727, #6554 ) ;
#52543=CARTESIAN_POINT ( 'NONE',  ( 0.000000000000000000, 0.000000000000000000, 0.000000000000000000 ) ) ;
#52675=DIRECTION ( 'NONE',  ( -0.9988488985473030768, 0.000000000000000000, 0.04796746679614544151 ) ) ;
#52759=ORIENTED_EDGE ( 'NONE', *, *, #15180, .T. ) ;
#52824=ORIENTED_EDGE ( 'NONE', *, *, #67854, .T. ) ;
#52853=DIRECTION ( 'NONE',  ( 0.000000000000000000, 0.000000000000000000, -1.000000000000000000 ) ) ;
#52862=CARTESIAN_POINT ( 'NONE',  ( 5.850262805259840881, 192.0000000000000000, -1.724042536399416514 ) ) ;
#52941=CARTESIAN_POINT ( 'NONE',  ( 9.850262805259839993, 192.0000000000000000, -1.724042536399416514 ) ) ;
#53200=ADVANCED_FACE ( 'NONE', ( #68520 ), #47737, .F. ) ;
#53236=EDGE_CURVE ( 'NONE', #23774, #19589, #68801, .T. ) ;
#53282=EDGE_CURVE ( 'NONE', #17365, #43631, #10118, .T. ) ;
#53348=EDGE_CURVE ( 'NONE', #32164, #22494, #5922, .T. ) ;
#53408=VERTEX_POINT ( 'NONE', #17466 ) ;
#53439=VERTEX_POINT ( 'NONE', #22404 ) ;
#53523=CARTESIAN_POINT ( 'NONE',  ( 5.850262805259839993, 200.0000000000000000, -1.724042536399416070 ) ) ;
#53571=EDGE_CURVE ( 'NONE', #22494, #53439, #9699, .T. ) ;
#53612=AXIS2_PLACEMENT_3D ( 'NONE', #61609, #52087, #68278 ) ;
#53700=LINE ( 'NONE', #32607, #53937 ) ;
#53705=CARTESIAN_POINT ( 'NONE',  ( -4.000000000000000000, 188.0000000000000000, 0.000000000000000000 ) ) ;
#53772=CARTESIAN_POINT ( 'NONE',  ( 5.737557066527558369, 192.0000000000000000, 2.275957463600585040 ) ) ;
#53790=PRODUCT_DEFINITION ( 'UNKNOWN', '', #25447, #32442 ) ;
#53937=VECTOR ( 'NONE', #38574, 1000.000000000000227 ) ;
#54154=ADVANCED_BREP_SHAPE_REPRESENTATION ( '', ( #40699, #66832 ), #11806 ) ;
#54241=ORIENTED_EDGE ( 'NONE', *, *, #47561, .F. ) ;
#54280=DIRECTION ( 'NONE',  ( -0.000000000000000000, -1.000000000000000000, -0.000000000000000000 ) ) ;
#54306=CARTESIAN_POINT ( 'NONE',  ( 0.000000000000000000, 70.00000000000000000, 0.000000000000000000 ) ) ;
#54482=DIRECTION ( 'NONE',  ( 0.000000000000000000, -1.000000000000000000, 0.000000000000000000 ) ) ;
#54727=DIRECTION ( 'NONE',  ( 0.000000000000000000, 1.000000000000000000, 0.000000000000000000 ) ) ;
#54768=EDGE_CURVE ( 'NONE', #43885, #20839, #25470, .T. ) ;
#54770=CIRCLE ( 'NONE', #55902, 10.00000000000000355 ) ;
#54785=VERTEX_POINT ( 'NONE', #58480 ) ;
#54866=DIRECTION ( 'NONE',  ( 0.000000000000000000, 0.000000000000000000, -1.000000000000000000 ) ) ;
#54885=ORIENTED_EDGE ( 'NONE', *, *, #41385, .T. ) ;
#54908=DIRECTION ( 'NONE',  ( 0.000000000000000000, 0.000000000000000000, -1.000000000000000000 ) ) ;
#55049=EDGE_CURVE ( 'NONE', #24494, #48193, #35234, .T. ) ;
#55289=CARTESIAN_POINT ( 'NONE',  ( -29.68020330876228030, 70.00000000000000000, 4.368699068434031219 ) ) ;
#55404=DIRECTION ( 'NONE',  ( -0.01289363347198224825, 0.000000000000000000, -0.9999168736529503443 ) ) ;
#55587=EDGE_CURVE ( 'NONE', #28455, #32766, #56093, .T. ) ;
#55598=AXIS2_PLACEMENT_3D ( 'NONE', #54306, #15663, #37111 ) ;
#55616=CARTESIAN_POINT ( 'NONE',  ( 0.000000000000000000, 70.00000000000000000, 0.000000000000000000 ) ) ;
#55697=CARTESIAN_POINT ( 'NONE',  ( -17.36794314067741496, 70.00000000000000000, 24.46128678263259815 ) ) ;
#55902=AXIS2_PLACEMENT_3D ( 'NONE', #60387, #65317, #17103 ) ;
#55912=DIRECTION ( 'NONE',  ( 0.000000000000000000, 1.000000000000000000, -0.000000000000000000 ) ) ;
#55959=DIRECTION ( 'NONE',  ( 0.000000000000000000, -0.000000000000000000, 1.000000000000000000 ) ) ;
#56043=CARTESIAN_POINT ( 'NONE',  ( 9.249622075198342230, 0.000000000000000000, 3.800590936420744193 ) ) ;
#56093=LINE ( 'NONE', #19489, #45416 ) ;
#56140=LINE ( 'NONE', #33659, #24027 ) ;
#56343=DIRECTION ( 'NONE',  ( 0.000000000000000000, 0.000000000000000000, -1.000000000000000000 ) ) ;
#56453=AXIS2_PLACEMENT_3D ( 'NONE', #17, #64385, #54866 ) ;
#56611=VECTOR ( 'NONE', #63995, 1000.000000000000000 ) ;
#56756=( LENGTH_UNIT ( ) NAMED_UNIT ( * ) SI_UNIT ( .MILLI., .METRE. ) );
#56783=DIRECTION ( 'NONE',  ( 0.000000000000000000, 1.000000000000000000, 0.000000000000000000 ) ) ;
#56956=PRODUCT_DEFINITION_SHAPE ( 'NONE', 'NONE',  #53790 ) ;
#57004=VERTEX_POINT ( 'NONE', #62603 ) ;
#57009=DIRECTION ( 'NONE',  ( 0.8890122540821405739, 0.000000000000000000, 0.4578834044730072383 ) ) ;
#57109=EDGE_CURVE ( 'NONE', #8643, #24463, #37925, .T. ) ;
#57318=CIRCLE ( 'NONE', #44957, 10.00000000000000000 ) ;
#57324=ADVANCED_FACE ( 'NONE', ( #5820 ), #59626, .T. ) ;
#57446=SURFACE_STYLE_USAGE ( .BOTH. , #51485 ) ;
#57536=CLOSED_SHELL ( 'NONE', ( #52521, #57324, #26442, #60915, #59800, #45273, #10960, #66572, #50205, #61468, #44133, #30328, #27709, #50825, #33030, #3559, #53200, #63894, #37408, #36053, #66792 ) ) ;
#57974=VECTOR ( 'NONE', #21094, 1000.000000000000000 ) ;
#58022=ORIENTED_EDGE ( 'NONE', *, *, #57109, .F. ) ;
#58088=DIRECTION ( 'NONE',  ( 0.000000000000000000, -1.000000000000000000, 0.000000000000000000 ) ) ;
#58225=DIRECTION ( 'NONE',  ( -0.000000000000000000, -1.000000000000000000, -0.000000000000000000 ) ) ;
#58313=DIRECTION ( 'NONE',  ( -0.000000000000000000, -1.000000000000000000, -0.000000000000000000 ) ) ;
#58381=VERTEX_POINT ( 'NONE', #66179 ) ;
#58479=DIRECTION ( 'NONE',  ( -1.000000000000000000, 0.000000000000000000, -0.000000000000000000 ) ) ;
#58480=CARTESIAN_POINT ( 'NONE',  ( 18.62350602913452846, 70.00000000000000000, 23.51946052065798298 ) ) ;
#58634=DIRECTION ( 'NONE',  ( -0.9988488985473030768, 0.000000000000000000, 0.04796746679614544151 ) ) ;
#58659=CIRCLE ( 'NONE', #67679, 30.00000000000000000 ) ;
#58886=ORIENTED_EDGE ( 'NONE', *, *, #18265, .T. ) ;
#58986=DIRECTION ( 'NONE',  ( 0.000000000000000000, 0.000000000000000000, -1.000000000000000000 ) ) ;
#59290=ORIENTED_EDGE ( 'NONE', *, *, #20480, .F. ) ;
#59463=EDGE_CURVE ( 'NONE', #18937, #16807, #26428, .T. ) ;
#59490=AXIS2_PLACEMENT_3D ( 'NONE', #2200, #24697, #56343 ) ;
#59626=CYLINDRICAL_SURFACE ( 'NONE', #27575, 10.00000000000000000 ) ;
#59767=CARTESIAN_POINT ( 'NONE',  ( 1.005827167100601827, 70.00000000000000000, -9.949286995052577964 ) ) ;
#59775=EDGE_CURVE ( 'NONE', #36732, #54785, #63332, .T. ) ;
#59779=EDGE_LOOP ( 'NONE', ( #34540, #52759, #59980, #46820 ) ) ;
#59800=ADVANCED_FACE ( 'NONE', ( #5947 ), #21783, .F. ) ;
#59933=CARTESIAN_POINT ( 'NONE',  ( 9.850262805259839993, 188.0000000000000000, -1.724042536399416070 ) ) ;
#59980=ORIENTED_EDGE ( 'NONE', *, *, #22370, .F. ) ;
#60168=ORIENTED_EDGE ( 'NONE', *, *, #6455, .F. ) ;
#60385=DIRECTION ( 'NONE',  ( 0.000000000000000000, 0.000000000000000000, -1.000000000000000000 ) ) ;
#60387=CARTESIAN_POINT ( 'NONE',  ( 0.000000000000000000, 0.000000000000000000, 0.000000000000000000 ) ) ;
#60439=PLANE ( 'NONE',  #19410 ) ;
#60484=LINE ( 'NONE', #6671, #450 ) ;
#60512=DIRECTION ( 'NONE',  ( -0.000000000000000000, 1.000000000000000000, -0.000000000000000000 ) ) ;
#60790=CYLINDRICAL_SURFACE ( 'NONE', #17075, 10.00000000000000000 ) ;
#60792=ORIENTED_EDGE ( 'NONE', *, *, #31278, .F. ) ;
#60819=EDGE_CURVE ( 'NONE', #53439, #24494, #47851, .T. ) ;
#60911=DIRECTION ( 'NONE',  ( 0.000000000000000000, -1.000000000000000000, 0.000000000000000000 ) ) ;
#60915=ADVANCED_FACE ( 'NONE', ( #14719 ), #35491, .T. ) ;
#60995=LINE ( 'NONE', #59933, #52003 ) ;
#61192=CIRCLE ( 'NONE', #3944, 10.00000000000000000 ) ;
#61468=ADVANCED_FACE ( 'NONE', ( #46557 ), #46210, .F. ) ;
#61527=EDGE_LOOP ( 'NONE', ( #37129, #46977, #25843, #2096 ) ) ;
#61580=DIRECTION ( 'NONE',  ( 0.000000000000000000, 1.000000000000000000, 0.000000000000000000 ) ) ;
#61609=CARTESIAN_POINT ( 'NONE',  ( 11.05669727962760085, 0.000000000000000000, -27.88815958909220782 ) ) ;
#61673=DIRECTION ( 'NONE',  ( 0.000000000000000000, -1.000000000000000000, 0.000000000000000000 ) ) ;
#61825=DIRECTION ( 'NONE',  ( 0.000000000000000000, -1.000000000000000000, 0.000000000000000000 ) ) ;
#61888=DIRECTION ( 'NONE',  ( -0.9988488985473030768, 0.000000000000000000, 0.04796746679614544151 ) ) ;
#61918=PLANE ( 'NONE',  #33209 ) ;
#61976=ORIENTED_EDGE ( 'NONE', *, *, #41608, .T. ) ;
#62033=CARTESIAN_POINT ( 'NONE',  ( -29.68020330876228030, 70.00000000000000000, 4.368699068434031219 ) ) ;
#62181=ORIENTED_EDGE ( 'NONE', *, *, #68391, .F. ) ;
#62236=DIRECTION ( 'NONE',  ( 0.000000000000000000, 0.000000000000000000, -1.000000000000000000 ) ) ;
#62242=CARTESIAN_POINT ( 'NONE',  ( -4.000000000000000000, 200.0000000000000000, 0.000000000000000000 ) ) ;
#62550=CARTESIAN_POINT ( 'NONE',  ( 1.005827167100601827, 0.000000000000000000, -9.949286995052577964 ) ) ;
#62581=CARTESIAN_POINT ( 'NONE',  ( -7.916219337932451694, 0.000000000000000000, 6.110112224316693208 ) ) ;
#62603=CARTESIAN_POINT ( 'NONE',  ( -12.50012419267789632, 70.00000000000000000, -27.27172336262651697 ) ) ;
#62682=ORIENTED_EDGE ( 'NONE', *, *, #49949, .F. ) ;
#62809=DIRECTION ( 'NONE',  ( 0.000000000000000000, -1.000000000000000000, 0.000000000000000000 ) ) ;
#62864=CIRCLE ( 'NONE', #35902, 10.00000000000000000 ) ;
#63277=ORIENTED_EDGE ( 'NONE', *, *, #32653, .F. ) ;
#63332=LINE ( 'NONE', #15142, #3990 ) ;
#63344=VECTOR ( 'NONE', #13577, 1000.000000000000000 ) ;
#63345=VECTOR ( 'NONE', #51069, 1000.000000000000000 ) ;
#63574=VECTOR ( 'NONE', #17348, 1000.000000000000000 ) ;
#63662=LINE ( 'NONE', #48471, #57974 ) ;
#63894=ADVANCED_FACE ( 'NONE', ( #34515 ), #2490, .T. ) ;
#63995=DIRECTION ( 'NONE',  ( 0.000000000000000000, -1.000000000000000000, 0.000000000000000000 ) ) ;
#64020=ORIENTED_EDGE ( 'NONE', *, *, #39021, .T. ) ;
#64208=DIRECTION ( 'NONE',  ( 0.000000000000000000, -1.000000000000000000, 0.000000000000000000 ) ) ;
#64367=CARTESIAN_POINT ( 'NONE',  ( -29.68020330876228385, 70.00000000000000000, 4.368699068434031219 ) ) ;
#64385=DIRECTION ( 'NONE',  ( 0.000000000000000000, -1.000000000000000000, 0.000000000000000000 ) ) ;
#64726=DIRECTION ( 'NONE',  ( -0.9999168736529502333, 0.000000000000000000, 0.01289363347198224652 ) ) ;
#65317=DIRECTION ( 'NONE',  ( 0.000000000000000000, -1.000000000000000000, 0.000000000000000000 ) ) ;
#65358=EDGE_CURVE ( 'NONE', #32164, #31926, #40862, .T. ) ;
#65385=EDGE_CURVE ( 'NONE', #1859, #17365, #30338, .T. ) ;
#65390=ORIENTED_EDGE ( 'NONE', *, *, #67854, .F. ) ;
#65605=ORIENTED_EDGE ( 'NONE', *, *, #47650, .F. ) ;
#65900=PRODUCT ( 'rotor', 'rotor', '', ( #69118 ) ) ;
#65988=PLANE ( 'NONE',  #50639 ) ;
#66179=CARTESIAN_POINT ( 'NONE',  ( 11.05669727962760085, 70.00000000000000000, -27.88815958909220782 ) ) ;
#66264=EDGE_LOOP ( 'NONE', ( #6088, #50328, #39663, #44208, #10688, #29992, #40818, #67222, #2584, #15042, #11175, #25576, #26749 ) ) ;
#66291=ORIENTED_EDGE ( 'NONE', *, *, #1209, .F. ) ;
#66572=ADVANCED_FACE ( 'NONE', ( #51778 ), #3584, .T. ) ;
#66791=DIRECTION ( 'NONE',  ( 0.000000000000000000, 1.000000000000000000, -0.000000000000000000 ) ) ;
#66792=ADVANCED_FACE ( 'NONE', ( #24629 ), #40105, .T. ) ;
#66832=AXIS2_PLACEMENT_3D ( 'NONE', #50530, #44558, #8319 ) ;
#66907=FACE_OUTER_BOUND ( 'NONE', #29313, .T. ) ;
#66932=DIRECTION ( 'NONE',  ( 0.000000000000000000, 0.000000000000000000, -1.000000000000000000 ) ) ;
#66987=UNCERTAINTY_MEASURE_WITH_UNIT (LENGTH_MEASURE( 1.000000000000000082E-05 ), #56756, 'distance_accuracy_value', 'NONE');
#67199=CARTESIAN_POINT ( 'NONE',  ( 0.000000000000000000, 192.0000000000000000, 0.000000000000000000 ) ) ;
#67222=ORIENTED_EDGE ( 'NONE', *, *, #3205, .T. ) ;
#67319=CARTESIAN_POINT ( 'NONE',  ( 8.113421703707349053, 0.000000000000000000, 5.845715376051984435 ) ) ;
#67367=ORIENTED_EDGE ( 'NONE', *, *, #53236, .T. ) ;
#67424=ORIENTED_EDGE ( 'NONE', *, *, #8268, .T. ) ;
#67603=DIRECTION ( 'NONE',  ( -0.000000000000000000, -1.000000000000000000, -0.000000000000000000 ) ) ;
#67679=AXIS2_PLACEMENT_3D ( 'NONE', #17892, #61825, #34773 ) ;
#67814=CARTESIAN_POINT ( 'NONE',  ( 0.000000000000000000, 0.000000000000000000, 0.000000000000000000 ) ) ;
#67854=EDGE_CURVE ( 'NONE', #54785, #24463, #309, .T. ) ;
#67880=VECTOR ( 'NONE', #37708, 1000.000000000000227 ) ;
#68258=ORIENTED_EDGE ( 'NONE', *, *, #13961, .T. ) ;
#68278=DIRECTION ( 'NONE',  ( 0.4887922226926451064, 0.000000000000000000, -0.8724002309921653486 ) ) ;
#68391=EDGE_CURVE ( 'NONE', #18937, #19589, #37021, .T. ) ;
#68520=FACE_OUTER_BOUND ( 'NONE', #17095, .T. ) ;
#68684=CARTESIAN_POINT ( 'NONE',  ( -9.119248870808011276, 0.000000000000000000, 4.103571619000548232 ) ) ;
#68775=SHAPE_DEFINITION_REPRESENTATION ( #56956, #36174 ) ;
#68801=CIRCLE ( 'NONE', #46367, 10.00000000000000000 ) ;
#68982=VECTOR ( 'NONE', #19639, 1000.000000000000000 ) ;
#69118=PRODUCT_CONTEXT ( 'NONE', #51611, 'mechanical' ) ;
#69176=CARTESIAN_POINT ( 'NONE',  ( -12.50012419267789632, 0.000000000000000000, -27.27172336262651697 ) ) ;
#69376=LINE ( 'NONE', #68684, #67880 ) ;
#69406=ORIENTED_EDGE ( 'NONE', *, *, #1209, .T. ) ;
#69410=EDGE_CURVE ( 'NONE', #7619, #8543, #31925, .T. ) ;
#69537=ORIENTED_EDGE ( 'NONE', *, *, #65358, .T. ) ;
ENDSEC;
END-ISO-10303-21;
